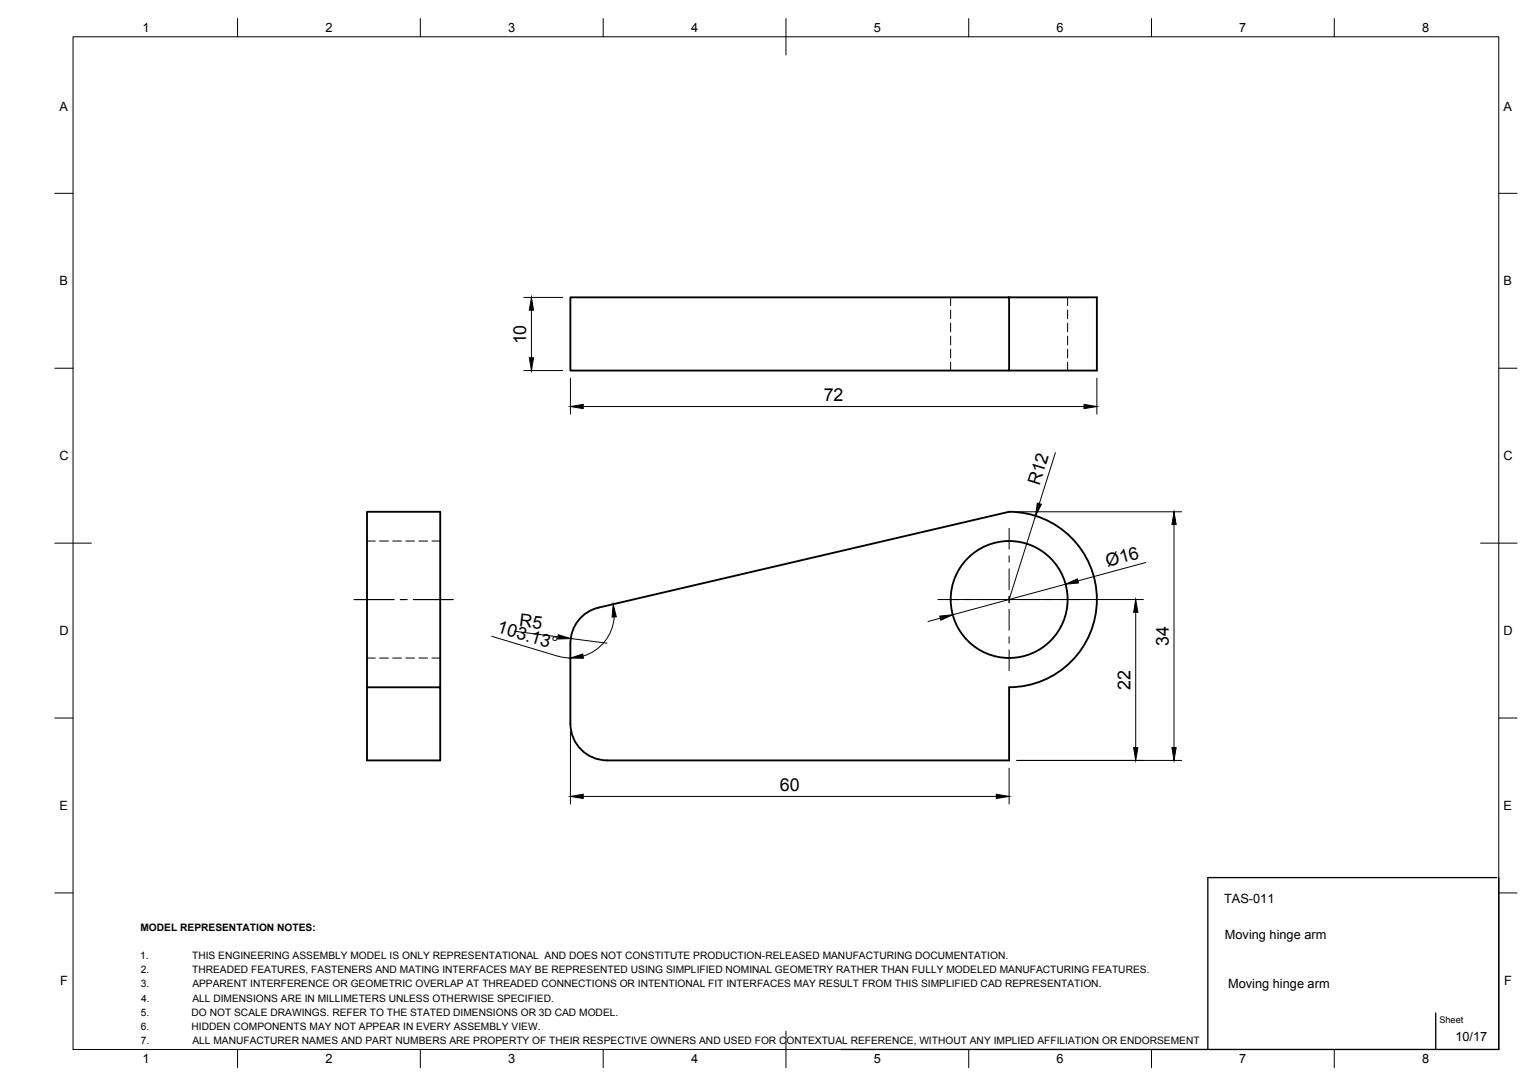
ISO-10303-21;
HEADER;
/* Generated by software containing ST-Developer
 * from STEP Tools, Inc. (www.steptools.com) 
 */

FILE_DESCRIPTION(
/* description */ (
'Independent manual bench leaf bending machine,200mm work width. Fabri
cated welded frame and folding leaf, repeated bushed and fully retaine
d hinge hardware, two handles with bonded grips, beveled clamping beam
 and modeledM12 clamp screws.2mm omitted-workpiece assembly reference 
gap, not a capacity claim. Native135deg hinge travel. Weld sizing, pro
duction fits, material condition, bending capacity, strength and life 
unassigned.'),
/* implementation_level */ '2;1');

FILE_NAME(
/* name */ 'Moving hinge arm.step',
/* time_stamp */ '2026-11-14T09:11:34-08:00',
/* author */ (''),
/* organization */ (''),
/* preprocessor_version */ 'ST-DEVELOPER v20.2',
/* originating_system */ 'Autodesk Translation Framework v15.17.0.0',
/* authorisation */ '');

FILE_SCHEMA (('AUTOMOTIVE_DESIGN { 1 0 10303 214 3 1 1 }'));
ENDSEC;

DATA;
#10=MECHANICAL_DESIGN_GEOMETRIC_PRESENTATION_REPRESENTATION('',(#455),#37701);
#419=SHAPE_REPRESENTATION_RELATIONSHIP('SRR','None',#37788,#437);
#437=ADVANCED_BREP_SHAPE_REPRESENTATION('',(#473),#37692);
#455=STYLED_ITEM('',(#37881),#473);
#473=MANIFOLD_SOLID_BREP('Body1',#4153);
#506=FACE_BOUND('',#1000,.T.);
#507=FACE_BOUND('',#1008,.T.);
#566=PLANE('',#4581);
#567=PLANE('',#4582);
#568=PLANE('',#4588);
#569=PLANE('',#4591);
#570=PLANE('',#4594);
#571=PLANE('',#4595);
#761=FACE_OUTER_BOUND('',#997,.T.);
#762=FACE_OUTER_BOUND('',#998,.T.);
#763=FACE_OUTER_BOUND('',#999,.T.);
#764=FACE_OUTER_BOUND('',#1001,.T.);
#765=FACE_OUTER_BOUND('',#1002,.T.);
#766=FACE_OUTER_BOUND('',#1003,.T.);
#767=FACE_OUTER_BOUND('',#1004,.T.);
#768=FACE_OUTER_BOUND('',#1005,.T.);
#769=FACE_OUTER_BOUND('',#1006,.T.);
#770=FACE_OUTER_BOUND('',#1007,.T.);
#997=EDGE_LOOP('',(#3625,#3626,#3627,#3628));
#998=EDGE_LOOP('',(#3629,#3630,#3631,#3632));
#999=EDGE_LOOP('',(#3633,#3634,#3635,#3636,#3637,#3638,#3639));
#1000=EDGE_LOOP('',(#3640));
#1001=EDGE_LOOP('',(#3641,#3642,#3643,#3644));
#1002=EDGE_LOOP('',(#3645,#3646,#3647,#3648));
#1003=EDGE_LOOP('',(#3649,#3650,#3651,#3652));
#1004=EDGE_LOOP('',(#3653,#3654,#3655,#3656));
#1005=EDGE_LOOP('',(#3657,#3658,#3659,#3660));
#1006=EDGE_LOOP('',(#3661,#3662,#3663,#3664));
#1007=EDGE_LOOP('',(#3665,#3666,#3667,#3668,#3669,#3670,#3671));
#1008=EDGE_LOOP('',(#3672));
#1250=LINE('',#37417,#1499);
#1251=LINE('',#37420,#1500);
#1252=LINE('',#37423,#1501);
#1253=LINE('',#37425,#1502);
#1254=LINE('',#37426,#1503);
#1255=LINE('',#37429,#1504);
#1256=LINE('',#37433,#1505);
#1257=LINE('',#37436,#1506);
#1258=LINE('',#37443,#1507);
#1259=LINE('',#37444,#1508);
#1260=LINE('',#37447,#1509);
#1261=LINE('',#37448,#1510);
#1262=LINE('',#37452,#1511);
#1263=LINE('',#37454,#1512);
#1264=LINE('',#37458,#1513);
#1265=LINE('',#37460,#1514);
#1499=VECTOR('',#5335,10.);
#1500=VECTOR('',#5338,10.);
#1501=VECTOR('',#5341,10.);
#1502=VECTOR('',#5342,10.);
#1503=VECTOR('',#5343,10.);
#1504=VECTOR('',#5346,10.);
#1505=VECTOR('',#5349,10.);
#1506=VECTOR('',#5352,10.);
#1507=VECTOR('',#5359,10.);
#1508=VECTOR('',#5360,10.);
#1509=VECTOR('',#5363,10.);
#1510=VECTOR('',#5364,10.);
#1511=VECTOR('',#5369,8.);
#1512=VECTOR('',#5372,10.);
#1513=VECTOR('',#5377,10.);
#1514=VECTOR('',#5380,10.);
#1603=CIRCLE('',#4579,5.);
#1604=CIRCLE('',#4580,5.);
#1605=CIRCLE('',#4583,5.);
#1606=CIRCLE('',#4584,12.);
#1607=CIRCLE('',#4585,8.);
#1608=CIRCLE('',#4587,5.);
#1609=CIRCLE('',#4590,8.);
#1610=CIRCLE('',#4593,12.);
#1991=VERTEX_POINT('',#37413);
#1992=VERTEX_POINT('',#37414);
#1993=VERTEX_POINT('',#37416);
#1994=VERTEX_POINT('',#37418);
#1995=VERTEX_POINT('',#37422);
#1996=VERTEX_POINT('',#37424);
#1997=VERTEX_POINT('',#37428);
#1998=VERTEX_POINT('',#37430);
#1999=VERTEX_POINT('',#37432);
#2000=VERTEX_POINT('',#37434);
#2001=VERTEX_POINT('',#37437);
#2002=VERTEX_POINT('',#37440);
#2003=VERTEX_POINT('',#37441);
#2004=VERTEX_POINT('',#37446);
#2005=VERTEX_POINT('',#37450);
#2006=VERTEX_POINT('',#37456);
#2546=EDGE_CURVE('',#1991,#1992,#1603,.T.);
#2547=EDGE_CURVE('',#1992,#1993,#1250,.T.);
#2548=EDGE_CURVE('',#1993,#1994,#1604,.T.);
#2549=EDGE_CURVE('',#1994,#1991,#1251,.T.);
#2550=EDGE_CURVE('',#1994,#1995,#1252,.T.);
#2551=EDGE_CURVE('',#1995,#1996,#1253,.T.);
#2552=EDGE_CURVE('',#1991,#1996,#1254,.T.);
#2553=EDGE_CURVE('',#1997,#1993,#1255,.T.);
#2554=EDGE_CURVE('',#1998,#1997,#1605,.T.);
#2555=EDGE_CURVE('',#1999,#1998,#1256,.T.);
#2556=EDGE_CURVE('',#2000,#1999,#1606,.T.);
#2557=EDGE_CURVE('',#1995,#2000,#1257,.T.);
#2558=EDGE_CURVE('',#2001,#2001,#1607,.T.);
#2559=EDGE_CURVE('',#2002,#2003,#1608,.T.);
#2560=EDGE_CURVE('',#2003,#1998,#1258,.T.);
#2561=EDGE_CURVE('',#1997,#2002,#1259,.T.);
#2562=EDGE_CURVE('',#2004,#2003,#1260,.T.);
#2563=EDGE_CURVE('',#1999,#2004,#1261,.T.);
#2564=EDGE_CURVE('',#2005,#2005,#1609,.T.);
#2565=EDGE_CURVE('',#2005,#2001,#1262,.T.);
#2566=EDGE_CURVE('',#2002,#1992,#1263,.T.);
#2567=EDGE_CURVE('',#2006,#2004,#1610,.T.);
#2568=EDGE_CURVE('',#2000,#2006,#1264,.T.);
#2569=EDGE_CURVE('',#1996,#2006,#1265,.T.);
#3625=ORIENTED_EDGE('',*,*,#2546,.T.);
#3626=ORIENTED_EDGE('',*,*,#2547,.T.);
#3627=ORIENTED_EDGE('',*,*,#2548,.T.);
#3628=ORIENTED_EDGE('',*,*,#2549,.T.);
#3629=ORIENTED_EDGE('',*,*,#2549,.F.);
#3630=ORIENTED_EDGE('',*,*,#2550,.T.);
#3631=ORIENTED_EDGE('',*,*,#2551,.T.);
#3632=ORIENTED_EDGE('',*,*,#2552,.F.);
#3633=ORIENTED_EDGE('',*,*,#2548,.F.);
#3634=ORIENTED_EDGE('',*,*,#2553,.F.);
#3635=ORIENTED_EDGE('',*,*,#2554,.F.);
#3636=ORIENTED_EDGE('',*,*,#2555,.F.);
#3637=ORIENTED_EDGE('',*,*,#2556,.F.);
#3638=ORIENTED_EDGE('',*,*,#2557,.F.);
#3639=ORIENTED_EDGE('',*,*,#2550,.F.);
#3640=ORIENTED_EDGE('',*,*,#2558,.T.);
#3641=ORIENTED_EDGE('',*,*,#2559,.T.);
#3642=ORIENTED_EDGE('',*,*,#2560,.T.);
#3643=ORIENTED_EDGE('',*,*,#2554,.T.);
#3644=ORIENTED_EDGE('',*,*,#2561,.T.);
#3645=ORIENTED_EDGE('',*,*,#2560,.F.);
#3646=ORIENTED_EDGE('',*,*,#2562,.F.);
#3647=ORIENTED_EDGE('',*,*,#2563,.F.);
#3648=ORIENTED_EDGE('',*,*,#2555,.T.);
#3649=ORIENTED_EDGE('',*,*,#2564,.F.);
#3650=ORIENTED_EDGE('',*,*,#2565,.T.);
#3651=ORIENTED_EDGE('',*,*,#2558,.F.);
#3652=ORIENTED_EDGE('',*,*,#2565,.F.);
#3653=ORIENTED_EDGE('',*,*,#2547,.F.);
#3654=ORIENTED_EDGE('',*,*,#2566,.F.);
#3655=ORIENTED_EDGE('',*,*,#2561,.F.);
#3656=ORIENTED_EDGE('',*,*,#2553,.T.);
#3657=ORIENTED_EDGE('',*,*,#2556,.T.);
#3658=ORIENTED_EDGE('',*,*,#2563,.T.);
#3659=ORIENTED_EDGE('',*,*,#2567,.F.);
#3660=ORIENTED_EDGE('',*,*,#2568,.F.);
#3661=ORIENTED_EDGE('',*,*,#2557,.T.);
#3662=ORIENTED_EDGE('',*,*,#2568,.T.);
#3663=ORIENTED_EDGE('',*,*,#2569,.F.);
#3664=ORIENTED_EDGE('',*,*,#2551,.F.);
#3665=ORIENTED_EDGE('',*,*,#2546,.F.);
#3666=ORIENTED_EDGE('',*,*,#2552,.T.);
#3667=ORIENTED_EDGE('',*,*,#2569,.T.);
#3668=ORIENTED_EDGE('',*,*,#2567,.T.);
#3669=ORIENTED_EDGE('',*,*,#2562,.T.);
#3670=ORIENTED_EDGE('',*,*,#2559,.F.);
#3671=ORIENTED_EDGE('',*,*,#2566,.T.);
#3672=ORIENTED_EDGE('',*,*,#2564,.T.);
#3915=CYLINDRICAL_SURFACE('',#4578,5.);
#3916=CYLINDRICAL_SURFACE('',#4586,5.);
#3917=CYLINDRICAL_SURFACE('',#4589,8.);
#3918=CYLINDRICAL_SURFACE('',#4592,12.);
#4091=ADVANCED_FACE('',(#761),#3915,.T.);
#4092=ADVANCED_FACE('',(#762),#566,.T.);
#4093=ADVANCED_FACE('',(#763,#506),#567,.F.);
#4094=ADVANCED_FACE('',(#764),#3916,.T.);
#4095=ADVANCED_FACE('',(#765),#568,.T.);
#4096=ADVANCED_FACE('',(#766),#3917,.F.);
#4097=ADVANCED_FACE('',(#767),#569,.T.);
#4098=ADVANCED_FACE('',(#768),#3918,.T.);
#4099=ADVANCED_FACE('',(#769),#570,.T.);
#4100=ADVANCED_FACE('',(#770,#507),#571,.T.);
#4153=CLOSED_SHELL('',(#4091,#4092,#4093,#4094,#4095,#4096,#4097,#4098,
#4099,#4100));
#4577=AXIS2_PLACEMENT_3D('',#37411,#5329,#5330);
#4578=AXIS2_PLACEMENT_3D('',#37412,#5331,#5332);
#4579=AXIS2_PLACEMENT_3D('',#37415,#5333,#5334);
#4580=AXIS2_PLACEMENT_3D('',#37419,#5336,#5337);
#4581=AXIS2_PLACEMENT_3D('',#37421,#5339,#5340);
#4582=AXIS2_PLACEMENT_3D('',#37427,#5344,#5345);
#4583=AXIS2_PLACEMENT_3D('',#37431,#5347,#5348);
#4584=AXIS2_PLACEMENT_3D('',#37435,#5350,#5351);
#4585=AXIS2_PLACEMENT_3D('',#37438,#5353,#5354);
#4586=AXIS2_PLACEMENT_3D('',#37439,#5355,#5356);
#4587=AXIS2_PLACEMENT_3D('',#37442,#5357,#5358);
#4588=AXIS2_PLACEMENT_3D('',#37445,#5361,#5362);
#4589=AXIS2_PLACEMENT_3D('',#37449,#5365,#5366);
#4590=AXIS2_PLACEMENT_3D('',#37451,#5367,#5368);
#4591=AXIS2_PLACEMENT_3D('',#37453,#5370,#5371);
#4592=AXIS2_PLACEMENT_3D('',#37455,#5373,#5374);
#4593=AXIS2_PLACEMENT_3D('',#37457,#5375,#5376);
#4594=AXIS2_PLACEMENT_3D('',#37459,#5378,#5379);
#4595=AXIS2_PLACEMENT_3D('',#37461,#5381,#5382);
#5329=DIRECTION('axis',(0.,0.,1.));
#5330=DIRECTION('refdir',(1.,0.,0.));
#5331=DIRECTION('center_axis',(0.,1.,0.));
#5332=DIRECTION('ref_axis',(0.707106781186548,0.,-0.707106781186548));
#5333=DIRECTION('center_axis',(0.,-1.,0.));
#5334=DIRECTION('ref_axis',(0.707106781186548,0.,-0.707106781186548));
#5335=DIRECTION('',(0.,-1.,0.));
#5336=DIRECTION('center_axis',(0.,1.,0.));
#5337=DIRECTION('ref_axis',(0.707106781186548,0.,-0.707106781186548));
#5338=DIRECTION('',(0.,1.,0.));
#5339=DIRECTION('center_axis',(0.,0.,-1.));
#5340=DIRECTION('ref_axis',(-1.,0.,0.));
#5341=DIRECTION('',(-1.,0.,0.));
#5342=DIRECTION('',(0.,1.,0.));
#5343=DIRECTION('',(-1.,0.,0.));
#5344=DIRECTION('center_axis',(0.,1.,0.));
#5345=DIRECTION('ref_axis',(1.,0.,0.));
#5346=DIRECTION('',(0.,0.,-1.));
#5347=DIRECTION('center_axis',(0.,1.,0.));
#5348=DIRECTION('ref_axis',(0.78333569292048,0.,0.621598899771221));
#5349=DIRECTION('',(0.973841209741793,0.,-0.227229615606418));
#5350=DIRECTION('center_axis',(0.,1.,0.));
#5351=DIRECTION('ref_axis',(-3.70074341541719E-16,0.,-1.));
#5352=DIRECTION('',(0.,0.,1.));
#5353=DIRECTION('center_axis',(0.,1.,0.));
#5354=DIRECTION('ref_axis',(0.,0.,1.));
#5355=DIRECTION('center_axis',(0.,1.,0.));
#5356=DIRECTION('ref_axis',(0.78333569292048,0.,0.621598899771221));
#5357=DIRECTION('center_axis',(0.,-1.,0.));
#5358=DIRECTION('ref_axis',(0.78333569292048,0.,0.621598899771221));
#5359=DIRECTION('',(0.,-1.,0.));
#5360=DIRECTION('',(0.,1.,0.));
#5361=DIRECTION('center_axis',(0.227229615606418,0.,0.973841209741793));
#5362=DIRECTION('ref_axis',(0.973841209741793,0.,-0.227229615606418));
#5363=DIRECTION('',(0.973841209741793,0.,-0.227229615606418));
#5364=DIRECTION('',(0.,1.,0.));
#5365=DIRECTION('center_axis',(0.,-1.,0.));
#5366=DIRECTION('ref_axis',(0.,0.,1.));
#5367=DIRECTION('center_axis',(0.,-1.,0.));
#5368=DIRECTION('ref_axis',(0.,0.,1.));
#5369=DIRECTION('',(0.,-1.,0.));
#5370=DIRECTION('center_axis',(1.,0.,0.));
#5371=DIRECTION('ref_axis',(0.,0.,-1.));
#5372=DIRECTION('',(0.,0.,-1.));
#5373=DIRECTION('center_axis',(0.,1.,0.));
#5374=DIRECTION('ref_axis',(-3.70074341541719E-16,0.,-1.));
#5375=DIRECTION('center_axis',(0.,1.,0.));
#5376=DIRECTION('ref_axis',(-3.70074341541719E-16,0.,-1.));
#5377=DIRECTION('',(0.,1.,0.));
#5378=DIRECTION('center_axis',(-1.,0.,0.));
#5379=DIRECTION('ref_axis',(0.,0.,1.));
#5380=DIRECTION('',(0.,0.,1.));
#5381=DIRECTION('center_axis',(0.,1.,0.));
#5382=DIRECTION('ref_axis',(1.,0.,0.));
#37411=CARTESIAN_POINT('',(0.,0.,0.));
#37412=CARTESIAN_POINT('Origin',(55.,0.,25.));
#37413=CARTESIAN_POINT('',(55.,10.,20.));
#37414=CARTESIAN_POINT('',(60.,10.,25.));
#37415=CARTESIAN_POINT('Origin',(55.,10.,25.));
#37416=CARTESIAN_POINT('',(60.,0.,25.));
#37417=CARTESIAN_POINT('',(60.,0.,25.));
#37418=CARTESIAN_POINT('',(55.,0.,20.));
#37419=CARTESIAN_POINT('Origin',(55.,0.,25.));
#37420=CARTESIAN_POINT('',(55.,0.,20.));
#37421=CARTESIAN_POINT('Origin',(60.,0.,20.));
#37422=CARTESIAN_POINT('',(0.,0.,20.));
#37423=CARTESIAN_POINT('',(60.,0.,20.));
#37424=CARTESIAN_POINT('',(0.,10.,20.));
#37425=CARTESIAN_POINT('',(0.,0.,20.));
#37426=CARTESIAN_POINT('',(60.,10.,20.));
#37427=CARTESIAN_POINT('Origin',(24.,0.,37.));
#37428=CARTESIAN_POINT('',(60.,0.,36.0323593997502));
#37429=CARTESIAN_POINT('',(60.,0.,40.));
#37430=CARTESIAN_POINT('',(56.1361480780321,0.,40.9015654484592));
#37431=CARTESIAN_POINT('Origin',(55.,0.,36.0323593997502));
#37432=CARTESIAN_POINT('',(0.,0.,54.));
#37433=CARTESIAN_POINT('',(0.,0.,54.));
#37434=CARTESIAN_POINT('',(0.,0.,30.));
#37435=CARTESIAN_POINT('Origin',(4.44089209850063E-15,0.,42.));
#37436=CARTESIAN_POINT('',(0.,0.,20.));
#37437=CARTESIAN_POINT('',(9.79717439317883E-16,0.,34.));
#37438=CARTESIAN_POINT('Origin',(0.,0.,42.));
#37439=CARTESIAN_POINT('Origin',(55.,0.,36.0323593997502));
#37440=CARTESIAN_POINT('',(60.,10.,36.0323593997502));
#37441=CARTESIAN_POINT('',(56.1361480780321,10.,40.9015654484592));
#37442=CARTESIAN_POINT('Origin',(55.,10.,36.0323593997502));
#37443=CARTESIAN_POINT('',(56.1361480780321,0.,40.9015654484592));
#37444=CARTESIAN_POINT('',(60.,0.,36.0323593997502));
#37445=CARTESIAN_POINT('Origin',(0.,0.,54.));
#37446=CARTESIAN_POINT('',(0.,10.,54.));
#37447=CARTESIAN_POINT('',(0.,10.,54.));
#37448=CARTESIAN_POINT('',(0.,0.,54.));
#37449=CARTESIAN_POINT('Origin',(0.,5.,42.));
#37450=CARTESIAN_POINT('',(9.79717439317883E-16,10.,34.));
#37451=CARTESIAN_POINT('Origin',(0.,10.,42.));
#37452=CARTESIAN_POINT('',(9.79717439317883E-16,5.,34.));
#37453=CARTESIAN_POINT('Origin',(60.,0.,40.));
#37454=CARTESIAN_POINT('',(60.,10.,40.));
#37455=CARTESIAN_POINT('Origin',(4.44089209850063E-15,0.,42.));
#37456=CARTESIAN_POINT('',(0.,10.,30.));
#37457=CARTESIAN_POINT('Origin',(4.44089209850063E-15,10.,42.));
#37458=CARTESIAN_POINT('',(0.,0.,30.));
#37459=CARTESIAN_POINT('Origin',(0.,0.,20.));
#37460=CARTESIAN_POINT('',(0.,10.,20.));
#37461=CARTESIAN_POINT('Origin',(24.,10.,37.));
#37672=UNCERTAINTY_MEASURE_WITH_UNIT(LENGTH_MEASURE(0.01),#37702,
'DISTANCE_ACCURACY_VALUE',
'Maximum model space distance between geometric entities at asserted c
onnectivities');
#37681=UNCERTAINTY_MEASURE_WITH_UNIT(LENGTH_MEASURE(0.01),#37702,
'DISTANCE_ACCURACY_VALUE',
'Maximum model space distance between geometric entities at asserted c
onnectivities');
#37692=(
GEOMETRIC_REPRESENTATION_CONTEXT(3)
GLOBAL_UNCERTAINTY_ASSIGNED_CONTEXT((#37672))
GLOBAL_UNIT_ASSIGNED_CONTEXT((#37702,#37704,#37705))
REPRESENTATION_CONTEXT('','3D')
);
#37701=(
GEOMETRIC_REPRESENTATION_CONTEXT(3)
GLOBAL_UNCERTAINTY_ASSIGNED_CONTEXT((#37681))
GLOBAL_UNIT_ASSIGNED_CONTEXT((#37702,#37704,#37705))
REPRESENTATION_CONTEXT('','3D')
);
#37702=(
LENGTH_UNIT()
NAMED_UNIT(*)
SI_UNIT(.MILLI.,.METRE.)
);
#37704=(
NAMED_UNIT(*)
PLANE_ANGLE_UNIT()
SI_UNIT($,.RADIAN.)
);
#37705=(
NAMED_UNIT(*)
SI_UNIT($,.STERADIAN.)
SOLID_ANGLE_UNIT()
);
#37716=SHAPE_DEFINITION_REPRESENTATION(#37735,#37788);
#37735=PRODUCT_DEFINITION_SHAPE('',$,#37808);
#37788=SHAPE_REPRESENTATION('',(#4577),#37692);
#37797=PRODUCT_DEFINITION_CONTEXT('part definition',#37856,'design');
#37808=PRODUCT_DEFINITION('Moving hinge arm','Moving hinge arm',#37827,
#37797);
#37827=PRODUCT_DEFINITION_FORMATION('',$,#37868);
#37856=APPLICATION_CONTEXT(
'Core Data for Automotive Mechanical Design Process');
#37857=PRODUCT_CONTEXT('part definition',#37856,'mechanical');
#37868=PRODUCT('Moving hinge arm','Moving hinge arm',$,(#37857));
#37881=PRESENTATION_STYLE_ASSIGNMENT((#37889));
#37889=SURFACE_STYLE_USAGE(.BOTH.,#37897);
#37897=SURFACE_SIDE_STYLE('',(#37905));
#37905=SURFACE_STYLE_FILL_AREA(#37913);
#37913=FILL_AREA_STYLE('Opaque(81,175,227)',(#37921));
#37921=FILL_AREA_STYLE_COLOUR('Opaque(81,175,227)',#37929);
#37929=COLOUR_RGB('Opaque(81,175,227)',0.317647058823529,0.686274509803922,
0.890196078431372);
ENDSEC;
END-ISO-10303-21;
